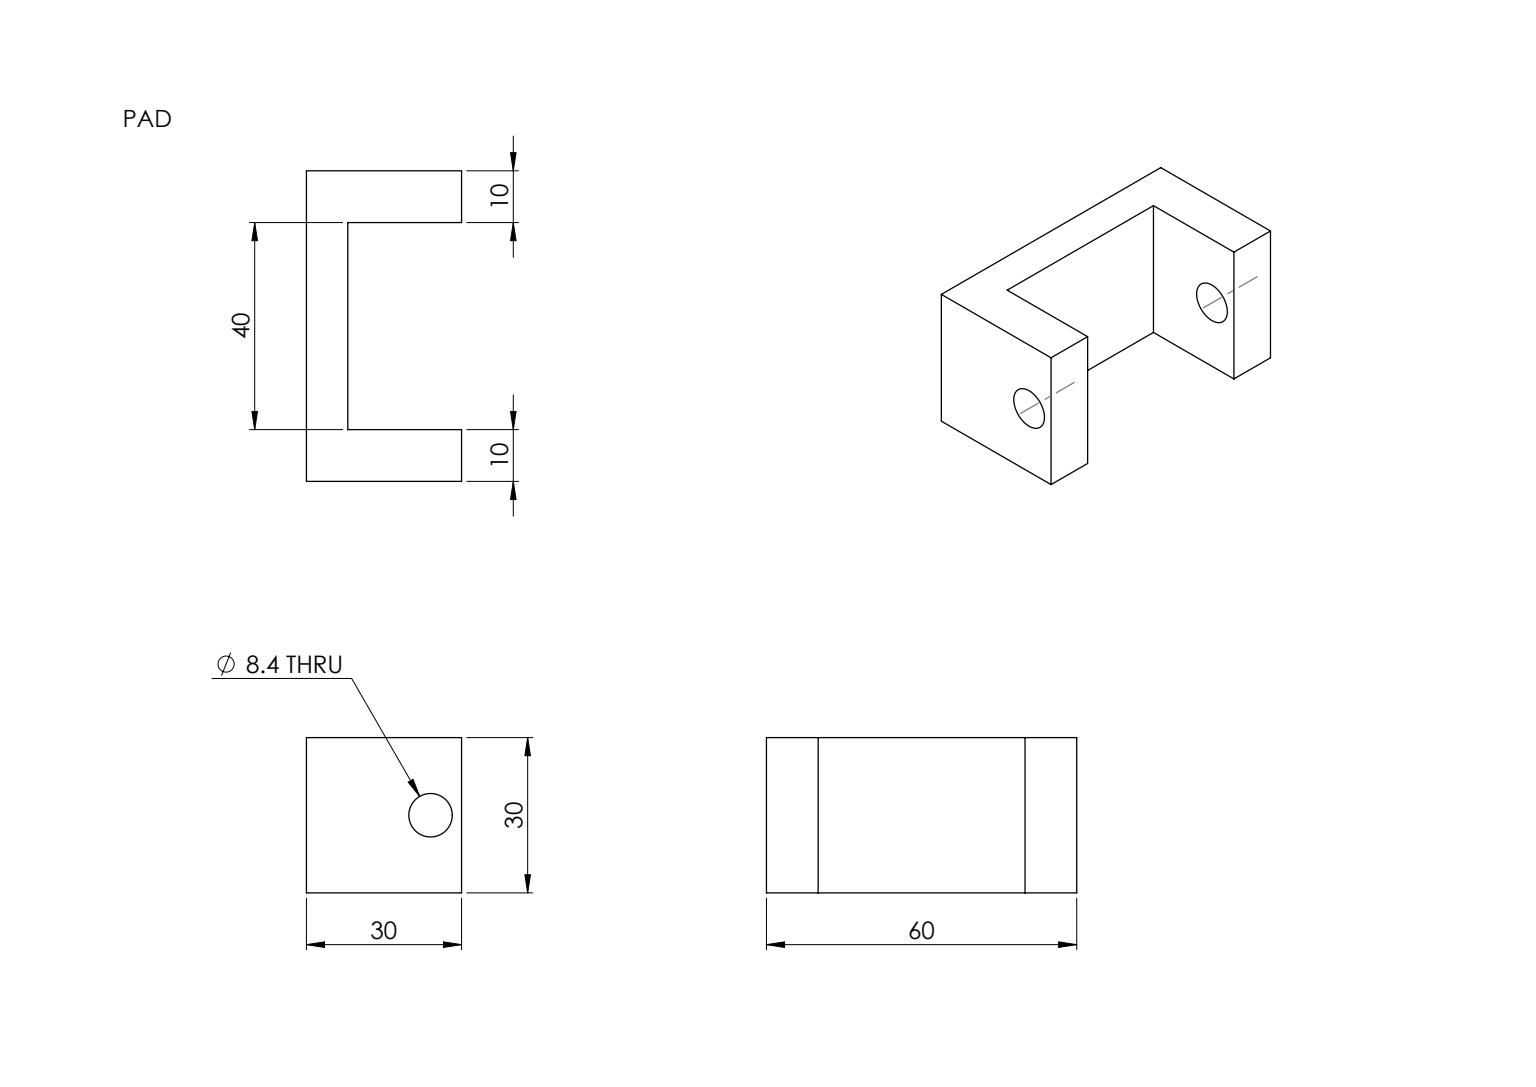
ISO-10303-21;
HEADER;
FILE_DESCRIPTION (('STEP AP214'),
    '1' );
FILE_NAME ('pad.step',
    '2026-10-08T07:58:12',
    ( '' ),
    ( '' ),
    'SwSTEP 2.0',
    'SolidWorks 2026',
    '' );
FILE_SCHEMA (( 'AUTOMOTIVE_DESIGN' ));
ENDSEC;

DATA;
#173=AXIS2_PLACEMENT_3D ( 'NONE', #29896, #20170, #1948 ) ;
#224=DIRECTION ( 'NONE',  ( -2.312964634635740985E-16, 1.000000000000000000, 0.000000000000000000 ) ) ;
#231=DIRECTION ( 'NONE',  ( -1.000000000000000000, 0.000000000000000000, -0.000000000000000000 ) ) ;
#282=APPLICATION_CONTEXT ( 'automotive_design' ) ;
#429=DIRECTION ( 'NONE',  ( -1.000000000000000000, 0.000000000000000000, 0.000000000000000000 ) ) ;
#437=CARTESIAN_POINT ( 'NONE',  ( 58.50000000000001421, -88.00000000000000000, -30.00000000000000000 ) ) ;
#514=PRODUCT_CONTEXT ( 'NONE', #30526, 'mechanical' ) ;
#517=DIRECTION ( 'NONE',  ( -0.000000000000000000, -0.000000000000000000, -1.000000000000000000 ) ) ;
#527=DIRECTION ( 'NONE',  ( 0.000000000000000000, -1.000000000000000000, 0.000000000000000000 ) ) ;
#576=VERTEX_POINT ( 'NONE', #31507 ) ;
#618=AXIS2_PLACEMENT_3D ( 'NONE', #25395, #27609, #7178 ) ;
#690=FACE_BOUND ( 'NONE', #27435, .T. ) ;
#731=AXIS2_PLACEMENT_3D ( 'NONE', #2930, #31053, #13311 ) ;
#790=UNCERTAINTY_MEASURE_WITH_UNIT (LENGTH_MEASURE( 1.000000000000000082E-05 ), #19917, 'distance_accuracy_value', 'NONE');
#873=DIRECTION ( 'NONE',  ( 0.000000000000000000, -1.000000000000000000, 0.000000000000000000 ) ) ;
#909=VECTOR ( 'NONE', #224, 1000.000000000000000 ) ;
#925=DIRECTION ( 'NONE',  ( 0.000000000000000000, 0.000000000000000000, -1.000000000000000000 ) ) ;
#942=LINE ( 'NONE', #11680, #28706 ) ;
#1001=( NAMED_UNIT ( * ) PLANE_ANGLE_UNIT ( ) SI_UNIT ( $, .RADIAN. ) );
#1029=LINE ( 'NONE', #22776, #23544 ) ;
#1286=ORIENTED_EDGE ( 'NONE', *, *, #8935, .F. ) ;
#1306=DIRECTION ( 'NONE',  ( 0.000000000000000000, 0.000000000000000000, -1.000000000000000000 ) ) ;
#1476=ADVANCED_FACE ( 'NONE', ( #27189 ), #19854, .F. ) ;
#1731=ORIENTED_EDGE ( 'NONE', *, *, #24172, .F. ) ;
#1733=CARTESIAN_POINT ( 'NONE',  ( 64.50000000000000000, 0.000000000000000000, 30.00000000000000000 ) ) ;
#1853=EDGE_CURVE ( 'NONE', #10439, #8233, #21818, .T. ) ;
#1857=MECHANICAL_DESIGN_GEOMETRIC_PRESENTATION_REPRESENTATION('',(#32884),#26900);
#1873=ORIENTED_EDGE ( 'NONE', *, *, #10837, .T. ) ;
#1914=LINE ( 'NONE', #1733, #4519 ) ;
#1938=DIRECTION ( 'NONE',  ( -2.312964634635740985E-16, 1.000000000000000000, 0.000000000000000000 ) ) ;
#1948=DIRECTION ( 'NONE',  ( -1.000000000000000000, 0.000000000000000000, 0.000000000000000000 ) ) ;
#2049=EDGE_LOOP ( 'NONE', ( #24718, #18953, #9756, #29271 ) ) ;
#2299=VERTEX_POINT ( 'NONE', #7168 ) ;
#2404=AXIS2_PLACEMENT_3D ( 'NONE', #8872, #11941, #4266 ) ;
#2667=LINE ( 'NONE', #7776, #31465 ) ;
#2693=CIRCLE ( 'NONE', #19527, 4.200000000000001954 ) ;
#2728=VERTEX_POINT ( 'NONE', #14113 ) ;
#2741=ADVANCED_BREP_SHAPE_REPRESENTATION ( '', ( #23155, #2404 ), #13844 ) ;
#2787=FACE_OUTER_BOUND ( 'NONE', #5141, .T. ) ;
#2913=VECTOR ( 'NONE', #28866, 1000.000000000000000 ) ;
#2915=CARTESIAN_POINT ( 'NONE',  ( 64.50000000000000000, 0.000000000000000000, -30.00000000000000000 ) ) ;
#2930=CARTESIAN_POINT ( 'NONE',  ( 64.50000000000000000, 0.000000000000000000, -30.00000000000000000 ) ) ;
#2935=ORIENTED_EDGE ( 'NONE', *, *, #16237, .F. ) ;
#2937=DIRECTION ( 'NONE',  ( -0.000000000000000000, -0.000000000000000000, -1.000000000000000000 ) ) ;
#2976=DIRECTION ( 'NONE',  ( -1.000000000000000000, 0.000000000000000000, 0.000000000000000000 ) ) ;
#3040=ORIENTED_EDGE ( 'NONE', *, *, #16988, .T. ) ;
#3111=ORIENTED_EDGE ( 'NONE', *, *, #30533, .F. ) ;
#3168=VERTEX_POINT ( 'NONE', #4394 ) ;
#3249=ORIENTED_EDGE ( 'NONE', *, *, #12805, .F. ) ;
#3324=ADVANCED_FACE ( 'NONE', ( #15125 ), #7471, .T. ) ;
#3411=DIRECTION ( 'NONE',  ( 0.000000000000000000, -1.000000000000000000, 0.000000000000000000 ) ) ;
#3539=CARTESIAN_POINT ( 'NONE',  ( 64.50000000000000000, -73.00000000000000000, -20.00000000000000000 ) ) ;
#3569=DIRECTION ( 'NONE',  ( -1.000000000000000000, 0.000000000000000000, -0.000000000000000000 ) ) ;
#3583=CYLINDRICAL_SURFACE ( 'NONE', #25243, 4.200000000000001954 ) ;
#3875=EDGE_CURVE ( 'NONE', #2728, #26702, #9594, .T. ) ;
#4080=( NAMED_UNIT ( * ) PLANE_ANGLE_UNIT ( ) SI_UNIT ( $, .RADIAN. ) );
#4152=ADVANCED_FACE ( 'NONE', ( #2787, #15720 ), #16050, .F. ) ;
#4238=FACE_BOUND ( 'NONE', #23300, .T. ) ;
#4250=AXIS2_PLACEMENT_3D ( 'NONE', #26142, #26305, #2976 ) ;
#4266=DIRECTION ( 'NONE',  ( 1.000000000000000000, 0.000000000000000000, 0.000000000000000000 ) ) ;
#4343=LINE ( 'NONE', #12347, #9410 ) ;
#4347=ORIENTED_EDGE ( 'NONE', *, *, #33290, .F. ) ;
#4378=EDGE_LOOP ( 'NONE', ( #20165, #13924, #27388, #19802 ) ) ;
#4394=CARTESIAN_POINT ( 'NONE',  ( 62.70000000000001705, -88.00000000000000000, 20.00000000000000000 ) ) ;
#4434=AXIS2_PLACEMENT_3D ( 'NONE', #13167, #31559, #231 ) ;
#4473=VERTEX_POINT ( 'NONE', #16883 ) ;
#4519=VECTOR ( 'NONE', #22349, 1000.000000000000000 ) ;
#4562=ADVANCED_FACE ( 'NONE', ( #22847 ), #32721, .F. ) ;
#4581=CARTESIAN_POINT ( 'NONE',  ( 64.50000000000000000, -73.00000000000000000, 20.00000000000000000 ) ) ;
#4635=DIRECTION ( 'NONE',  ( -0.000000000000000000, -0.000000000000000000, -1.000000000000000000 ) ) ;
#4744=ADVANCED_FACE ( 'NONE', ( #33061 ), #17222, .T. ) ;
#4781=AXIS2_PLACEMENT_3D ( 'NONE', #9687, #19741, #6970 ) ;
#4857=CARTESIAN_POINT ( 'NONE',  ( 4.764707147349631625E-14, -103.0000000000000284, 20.00000000000000000 ) ) ;
#5031=DIRECTION ( 'NONE',  ( -0.000000000000000000, -0.000000000000000000, -1.000000000000000000 ) ) ;
#5041=LINE ( 'NONE', #7432, #22790 ) ;
#5141=EDGE_LOOP ( 'NONE', ( #18509, #5550, #27056, #19591 ) ) ;
#5167=LINE ( 'NONE', #17775, #11213 ) ;
#5313=ORIENTED_EDGE ( 'NONE', *, *, #3875, .T. ) ;
#5478=FACE_OUTER_BOUND ( 'NONE', #15118, .T. ) ;
#5512=EDGE_LOOP ( 'NONE', ( #20983, #9749, #20862, #21763 ) ) ;
#5550=ORIENTED_EDGE ( 'NONE', *, *, #1853, .F. ) ;
#5623=EDGE_CURVE ( 'NONE', #4473, #30739, #9974, .T. ) ;
#5762=VERTEX_POINT ( 'NONE', #17800 ) ;
#5763=LINE ( 'NONE', #8339, #17293 ) ;
#5804=ORIENTED_EDGE ( 'NONE', *, *, #7261, .T. ) ;
#5983=EDGE_CURVE ( 'NONE', #8169, #8276, #19476, .T. ) ;
#6103=SHAPE_DEFINITION_REPRESENTATION ( #24933, #12832 ) ;
#6268=ORIENTED_EDGE ( 'NONE', *, *, #33328, .F. ) ;
#6393=LINE ( 'NONE', #11510, #11291 ) ;
#6521=CIRCLE ( 'NONE', #14123, 4.200000000000001954 ) ;
#6734=DIRECTION ( 'NONE',  ( 2.312964634635740985E-16, -1.000000000000000000, 0.000000000000000000 ) ) ;
#6750=VECTOR ( 'NONE', #517, 1000.000000000000000 ) ;
#6970=DIRECTION ( 'NONE',  ( 1.000000000000000000, 0.000000000000000000, 0.000000000000000000 ) ) ;
#6994=EDGE_CURVE ( 'NONE', #13849, #25466, #5041, .T. ) ;
#7168=CARTESIAN_POINT ( 'NONE',  ( 34.49999999999999289, -72.99999999999998579, 30.00000000000000000 ) ) ;
#7178=DIRECTION ( 'NONE',  ( 1.000000000000000000, 0.000000000000000000, 0.000000000000000000 ) ) ;
#7248=ORIENTED_EDGE ( 'NONE', *, *, #14578, .T. ) ;
#7261=EDGE_CURVE ( 'NONE', #13192, #9072, #2693, .T. ) ;
#7432=CARTESIAN_POINT ( 'NONE',  ( 124.9999999999999716, -73.00000000000002842, -20.00000000000000000 ) ) ;
#7471=PLANE ( 'NONE',  #25623 ) ;
#7600=CARTESIAN_POINT ( 'NONE',  ( 34.49999999999999289, -72.99999999999998579, 30.00000000000000000 ) ) ;
#7609=CARTESIAN_POINT ( 'NONE',  ( 42.49999999999999289, -72.99999999999998579, -20.00000000000000000 ) ) ;
#7633=DIRECTION ( 'NONE',  ( -0.000000000000000000, -0.000000000000000000, 1.000000000000000000 ) ) ;
#7739=AXIS2_PLACEMENT_3D ( 'NONE', #17395, #30007, #20287 ) ;
#7761=LINE ( 'NONE', #23428, #2913 ) ;
#7776=CARTESIAN_POINT ( 'NONE',  ( 64.50000000000000000, -73.00000000000000000, 30.00000000000000000 ) ) ;
#7879=VERTEX_POINT ( 'NONE', #26448 ) ;
#7921=DIRECTION ( 'NONE',  ( 1.000000000000000000, -4.625929269271484928E-16, 0.000000000000000000 ) ) ;
#8163=AXIS2_PLACEMENT_3D ( 'NONE', #19746, #27412, #3569 ) ;
#8169=VERTEX_POINT ( 'NONE', #9396 ) ;
#8233=VERTEX_POINT ( 'NONE', #19792 ) ;
#8276=VERTEX_POINT ( 'NONE', #28478 ) ;
#8339=CARTESIAN_POINT ( 'NONE',  ( 42.50000000000000000, -103.0000000000000142, -51.04834939252008041 ) ) ;
#8376=DIRECTION ( 'NONE',  ( -1.000000000000000000, 0.000000000000000000, 0.000000000000000000 ) ) ;
#8538=CARTESIAN_POINT ( 'NONE',  ( -3.376928366568182163E-14, -72.99999999999997158, 20.00000000000000000 ) ) ;
#8675=LINE ( 'NONE', #19067, #6750 ) ;
#8699=FACE_OUTER_BOUND ( 'NONE', #20171, .T. ) ;
#8824=( NAMED_UNIT ( * ) SI_UNIT ( $, .STERADIAN. ) SOLID_ANGLE_UNIT ( ) );
#8872=CARTESIAN_POINT ( 'NONE',  ( 0.000000000000000000, 0.000000000000000000, 0.000000000000000000 ) ) ;
#8879=ADVANCED_FACE ( 'NONE', ( #4238, #19581 ), #17018, .F. ) ;
#8935=EDGE_CURVE ( 'NONE', #8276, #8169, #6521, .T. ) ;
#9061=LINE ( 'NONE', #32909, #18707 ) ;
#9072=VERTEX_POINT ( 'NONE', #15767 ) ;
#9151=VERTEX_POINT ( 'NONE', #16768 ) ;
#9362=ORIENTED_EDGE ( 'NONE', *, *, #12805, .T. ) ;
#9396=CARTESIAN_POINT ( 'NONE',  ( 62.70000000000001705, -88.00000000000000000, -30.00000000000000000 ) ) ;
#9402=EDGE_CURVE ( 'NONE', #27639, #28972, #27107, .T. ) ;
#9410=VECTOR ( 'NONE', #20356, 1000.000000000000000 ) ;
#9434=VECTOR ( 'NONE', #3411, 1000.000000000000000 ) ;
#9594=LINE ( 'NONE', #28169, #16391 ) ;
#9672=( NAMED_UNIT ( * ) SI_UNIT ( $, .STERADIAN. ) SOLID_ANGLE_UNIT ( ) );
#9687=CARTESIAN_POINT ( 'NONE',  ( 58.50000000000001421, -88.00000000000000000, 30.00000000000000000 ) ) ;
#9707=PRODUCT ( 'pad', 'pad', '', ( #514 ) ) ;
#9749=ORIENTED_EDGE ( 'NONE', *, *, #15399, .F. ) ;
#9756=ORIENTED_EDGE ( 'NONE', *, *, #30533, .T. ) ;
#9836=CARTESIAN_POINT ( 'NONE',  ( 4.764707147349631625E-14, -103.0000000000000284, 30.00000000000000000 ) ) ;
#9850=CARTESIAN_POINT ( 'NONE',  ( 34.49999999999997868, 7.979727989493303168E-15, 30.00000000000000000 ) ) ;
#9851=PRESENTATION_STYLE_ASSIGNMENT (( #25517 ) ) ;
#9916=LINE ( 'NONE', #23373, #11098 ) ;
#9974=LINE ( 'NONE', #4857, #31993 ) ;
#10163=DIRECTION ( 'NONE',  ( -0.000000000000000000, -0.000000000000000000, -1.000000000000000000 ) ) ;
#10168=EDGE_CURVE ( 'NONE', #21673, #30739, #5763, .T. ) ;
#10180=VERTEX_POINT ( 'NONE', #21603 ) ;
#10439=VERTEX_POINT ( 'NONE', #14616 ) ;
#10563=ORIENTED_EDGE ( 'NONE', *, *, #15365, .F. ) ;
#10644=ADVANCED_FACE ( 'NONE', ( #28749 ), #31137, .T. ) ;
#10664=DIRECTION ( 'NONE',  ( 1.000000000000000000, -4.625929269271484928E-16, 0.000000000000000000 ) ) ;
#10691=DIRECTION ( 'NONE',  ( -1.000000000000000000, 0.000000000000000000, 0.000000000000000000 ) ) ;
#10759=CARTESIAN_POINT ( 'NONE',  ( 0.000000000000000000, 0.000000000000000000, -30.00000000000000000 ) ) ;
#10761=ADVANCED_FACE ( 'NONE', ( #15956 ), #26184, .T. ) ;
#10837=EDGE_CURVE ( 'NONE', #3168, #9151, #13223, .T. ) ;
#10927=DIRECTION ( 'NONE',  ( -1.000000000000000000, 0.000000000000000000, -0.000000000000000000 ) ) ;
#10940=LINE ( 'NONE', #23876, #16445 ) ;
#11052=ORIENTED_EDGE ( 'NONE', *, *, #18559, .F. ) ;
#11057=VECTOR ( 'NONE', #13458, 1000.000000000000000 ) ;
#11098=VECTOR ( 'NONE', #4635, 1000.000000000000000 ) ;
#11213=VECTOR ( 'NONE', #1938, 1000.000000000000000 ) ;
#11291=VECTOR ( 'NONE', #29908, 1000.000000000000000 ) ;
#11348=ORIENTED_EDGE ( 'NONE', *, *, #28931, .T. ) ;
#11427=EDGE_LOOP ( 'NONE', ( #17978, #32147, #14905, #2935, #25416, #24673, #1731, #4347 ) ) ;
#11461=ORIENTED_EDGE ( 'NONE', *, *, #33328, .T. ) ;
#11510=CARTESIAN_POINT ( 'NONE',  ( 124.9999999999999716, -73.00000000000002842, -30.00000000000000000 ) ) ;
#11680=CARTESIAN_POINT ( 'NONE',  ( 42.49999999999998579, 9.830099697201894772E-15, 20.00000000000000000 ) ) ;
#11941=DIRECTION ( 'NONE',  ( 0.000000000000000000, 0.000000000000000000, 1.000000000000000000 ) ) ;
#12002=CARTESIAN_POINT ( 'NONE',  ( 58.50000000000001421, -88.00000000000000000, -30.00000000000000000 ) ) ;
#12160=CARTESIAN_POINT ( 'NONE',  ( 42.49999999999999289, -103.0000000000000142, -20.00000000000000000 ) ) ;
#12307=CIRCLE ( 'NONE', #21020, 4.200000000000001954 ) ;
#12314=CLOSED_SHELL ( 'NONE', ( #19715, #4562, #4152, #10644, #23936, #10761, #3324, #15148, #4744, #19588, #22933, #8879, #1476, #17501 ) ) ;
#12336=STYLED_ITEM ( 'NONE', ( #14469 ), #23155 ) ;
#12347=CARTESIAN_POINT ( 'NONE',  ( 62.70000000000001705, -88.00000000000000000, -30.00000000000000000 ) ) ;
#12474=ORIENTED_EDGE ( 'NONE', *, *, #12848, .T. ) ;
#12573=DIRECTION ( 'NONE',  ( -1.000000000000000000, 4.625929269271484928E-16, 0.000000000000000000 ) ) ;
#12662=DIRECTION ( 'NONE',  ( 0.000000000000000000, 0.000000000000000000, -1.000000000000000000 ) ) ;
#12742=DIRECTION ( 'NONE',  ( -1.000000000000000000, -2.312964634635740985E-16, 0.000000000000000000 ) ) ;
#12744=( LENGTH_UNIT ( ) NAMED_UNIT ( * ) SI_UNIT ( .MILLI., .METRE. ) );
#12805=EDGE_CURVE ( 'NONE', #9151, #7879, #16672, .T. ) ;
#12832=SHAPE_REPRESENTATION ( 'pad', ( #2404 ), #13844 ) ;
#12848=EDGE_CURVE ( 'NONE', #13192, #8276, #8675, .T. ) ;
#12936=ORIENTED_EDGE ( 'NONE', *, *, #10837, .F. ) ;
#13063=ORIENTED_EDGE ( 'NONE', *, *, #5983, .T. ) ;
#13162=CARTESIAN_POINT ( 'NONE',  ( 34.49999999999998579, -2.093232994345345860E-14, -30.00000000000000000 ) ) ;
#13167=CARTESIAN_POINT ( 'NONE',  ( 0.000000000000000000, 0.000000000000000000, 30.00000000000000000 ) ) ;
#13192=VERTEX_POINT ( 'NONE', #31318 ) ;
#13223=CIRCLE ( 'NONE', #25753, 4.200000000000001954 ) ;
#13307=UNCERTAINTY_MEASURE_WITH_UNIT (LENGTH_MEASURE( 1.000000000000000082E-05 ), #32499, 'distance_accuracy_value', 'NONE');
#13311=DIRECTION ( 'NONE',  ( 0.000000000000000000, 0.000000000000000000, 1.000000000000000000 ) ) ;
#13458=DIRECTION ( 'NONE',  ( 0.000000000000000000, 0.000000000000000000, 1.000000000000000000 ) ) ;
#13482=ORIENTED_EDGE ( 'NONE', *, *, #5623, .T. ) ;
#13525=VECTOR ( 'NONE', #16707, 1000.000000000000000 ) ;
#13630=DIRECTION ( 'NONE',  ( 0.000000000000000000, 0.000000000000000000, -1.000000000000000000 ) ) ;
#13676=VERTEX_POINT ( 'NONE', #19358 ) ;
#13680=EDGE_LOOP ( 'NONE', ( #32271, #17127, #30068, #7248 ) ) ;
#13750=CIRCLE ( 'NONE', #173, 4.200000000000001954 ) ;
#13785=DIRECTION ( 'NONE',  ( -0.000000000000000000, -0.000000000000000000, 1.000000000000000000 ) ) ;
#13844=( GEOMETRIC_REPRESENTATION_CONTEXT ( 3 ) GLOBAL_UNCERTAINTY_ASSIGNED_CONTEXT ( ( #13307 ) ) GLOBAL_UNIT_ASSIGNED_CONTEXT ( ( #32499, #1001, #8824 ) ) REPRESENTATION_CONTEXT ( 'NONE', 'WORKASPACE' ) );
#13849=VERTEX_POINT ( 'NONE', #7609 ) ;
#13888=ORIENTED_EDGE ( 'NONE', *, *, #3875, .F. ) ;
#13924=ORIENTED_EDGE ( 'NONE', *, *, #31036, .F. ) ;
#14110=FILL_AREA_STYLE_COLOUR ( '', #16538 ) ;
#14113=CARTESIAN_POINT ( 'NONE',  ( 64.50000000000000000, -103.0000000000000000, -30.00000000000000000 ) ) ;
#14123=AXIS2_PLACEMENT_3D ( 'NONE', #437, #21048, #14973 ) ;
#14303=SURFACE_SIDE_STYLE ('',( #17371 ) ) ;
#14375=CARTESIAN_POINT ( 'NONE',  ( 42.50000000000000000, -103.0000000000000142, 20.00000000000000355 ) ) ;
#14396=DIRECTION ( 'NONE',  ( -0.000000000000000000, -0.000000000000000000, -1.000000000000000000 ) ) ;
#14469=PRESENTATION_STYLE_ASSIGNMENT (( #24704 ) ) ;
#14533=EDGE_CURVE ( 'NONE', #28972, #4473, #10940, .T. ) ;
#14578=EDGE_CURVE ( 'NONE', #10439, #4473, #21316, .T. ) ;
#14616=CARTESIAN_POINT ( 'NONE',  ( 64.50000000000000000, -103.0000000000000000, 30.00000000000000000 ) ) ;
#14759=DIRECTION ( 'NONE',  ( 4.625929269271485914E-16, -1.000000000000000000, 0.000000000000000000 ) ) ;
#14802=ORIENTED_EDGE ( 'NONE', *, *, #7261, .F. ) ;
#14806=( NAMED_UNIT ( * ) SI_UNIT ( $, .STERADIAN. ) SOLID_ANGLE_UNIT ( ) );
#14905=ORIENTED_EDGE ( 'NONE', *, *, #9402, .F. ) ;
#14973=DIRECTION ( 'NONE',  ( -1.000000000000000000, 0.000000000000000000, 0.000000000000000000 ) ) ;
#15099=AXIS2_PLACEMENT_3D ( 'NONE', #18525, #31791, #19183 ) ;
#15104=DIRECTION ( 'NONE',  ( 1.000000000000000000, 4.625929269271485914E-16, 0.000000000000000000 ) ) ;
#15118=EDGE_LOOP ( 'NONE', ( #26429, #13888, #3111, #28199 ) ) ;
#15125=FACE_OUTER_BOUND ( 'NONE', #11427, .T. ) ;
#15148=ADVANCED_FACE ( 'NONE', ( #19857, #33154 ), #27523, .T. ) ;
#15365=EDGE_CURVE ( 'NONE', #9072, #13192, #13750, .T. ) ;
#15399=EDGE_CURVE ( 'NONE', #26702, #21673, #22561, .T. ) ;
#15467=SURFACE_SIDE_STYLE ('',( #17681 ) ) ;
#15629=CARTESIAN_POINT ( 'NONE',  ( -3.376928366568182163E-14, -72.99999999999997158, 30.00000000000000000 ) ) ;
#15640=EDGE_CURVE ( 'NONE', #2728, #5762, #18292, .T. ) ;
#15720=FACE_BOUND ( 'NONE', #17974, .T. ) ;
#15732=DIRECTION ( 'NONE',  ( -1.000000000000000000, -4.625929269271485914E-16, 0.000000000000000000 ) ) ;
#15767=CARTESIAN_POINT ( 'NONE',  ( 62.70000000000001705, -88.00000000000000000, -20.00000000000000000 ) ) ;
#15866=PLANE ( 'NONE',  #731 ) ;
#15956=FACE_OUTER_BOUND ( 'NONE', #13680, .T. ) ;
#16050=PLANE ( 'NONE',  #4434 ) ;
#16071=LINE ( 'NONE', #20693, #22490 ) ;
#16115=AXIS2_PLACEMENT_3D ( 'NONE', #10759, #13630, #10927 ) ;
#16156=DIRECTION ( 'NONE',  ( 0.000000000000000000, 0.000000000000000000, 1.000000000000000000 ) ) ;
#16237=EDGE_CURVE ( 'NONE', #13849, #27639, #9061, .T. ) ;
#16391=VECTOR ( 'NONE', #20157, 1000.000000000000000 ) ;
#16433=EDGE_CURVE ( 'NONE', #8233, #5762, #9916, .T. ) ;
#16445=VECTOR ( 'NONE', #873, 1000.000000000000000 ) ;
#16538=COLOUR_RGB ( '', 0.09019608, 0.27058824, 0.51372549) ;
#16672=LINE ( 'NONE', #27069, #20914 ) ;
#16707=DIRECTION ( 'NONE',  ( -1.000000000000000000, -4.625929269271485914E-16, 0.000000000000000000 ) ) ;
#16768=CARTESIAN_POINT ( 'NONE',  ( 54.30000000000001137, -88.00000000000000000, 20.00000000000000000 ) ) ;
#16883=CARTESIAN_POINT ( 'NONE',  ( 64.50000000000000000, -103.0000000000000000, 20.00000000000000000 ) ) ;
#16988=EDGE_CURVE ( 'NONE', #21673, #13849, #1029, .T. ) ;
#17018=PLANE ( 'NONE',  #8163 ) ;
#17027=FILL_AREA_STYLE ('',( #27420 ) ) ;
#17105=CARTESIAN_POINT ( 'NONE',  ( 58.50000000000001421, -88.00000000000000000, 20.00000000000000000 ) ) ;
#17119=FACE_OUTER_BOUND ( 'NONE', #23530, .T. ) ;
#17127=ORIENTED_EDGE ( 'NONE', *, *, #29739, .F. ) ;
#17166=ORIENTED_EDGE ( 'NONE', *, *, #5983, .F. ) ;
#17222=PLANE ( 'NONE',  #7739 ) ;
#17286=PRODUCT_DEFINITION ( 'UNKNOWN', '', #26254, #18513 ) ;
#17293=VECTOR ( 'NONE', #16156, 1000.000000000000000 ) ;
#17308=DIRECTION ( 'NONE',  ( -1.000000000000000000, 0.000000000000000000, -0.000000000000000000 ) ) ;
#17371=SURFACE_STYLE_FILL_AREA ( #17027 ) ;
#17395=CARTESIAN_POINT ( 'NONE',  ( 42.49999999999999289, -72.99999999999998579, -51.04834939252008041 ) ) ;
#17501=ADVANCED_FACE ( 'NONE', ( #17119 ), #33297, .F. ) ;
#17550=AXIS2_PLACEMENT_3D ( 'NONE', #22412, #1306, #17308 ) ;
#17619=DIRECTION ( 'NONE',  ( -1.000000000000000000, -4.625929269271485914E-16, 0.000000000000000000 ) ) ;
#17680=DIRECTION ( 'NONE',  ( 2.312964634635740985E-16, -1.000000000000000000, 0.000000000000000000 ) ) ;
#17681=SURFACE_STYLE_FILL_AREA ( #24504 ) ;
#17775=CARTESIAN_POINT ( 'NONE',  ( 34.49999999999997868, 7.979727989493303168E-15, 30.00000000000000000 ) ) ;
#17800=CARTESIAN_POINT ( 'NONE',  ( 34.50000000000000000, -103.0000000000000142, -30.00000000000000000 ) ) ;
#17974=EDGE_LOOP ( 'NONE', ( #20146, #24747 ) ) ;
#17978=ORIENTED_EDGE ( 'NONE', *, *, #18891, .T. ) ;
#18084=EDGE_LOOP ( 'NONE', ( #33426, #31262, #28653, #3040 ) ) ;
#18266=EDGE_CURVE ( 'NONE', #576, #10439, #1914, .T. ) ;
#18292=LINE ( 'NONE', #33459, #21359 ) ;
#18386=ORIENTED_EDGE ( 'NONE', *, *, #21820, .F. ) ;
#18501=ORIENTED_EDGE ( 'NONE', *, *, #24317, .F. ) ;
#18509=ORIENTED_EDGE ( 'NONE', *, *, #21939, .F. ) ;
#18513=PRODUCT_DEFINITION_CONTEXT ( 'detailed design', #282, 'design' ) ;
#18525=CARTESIAN_POINT ( 'NONE',  ( 64.50000000000000000, 0.000000000000000000, 30.00000000000000000 ) ) ;
#18559=EDGE_CURVE ( 'NONE', #9072, #8169, #4343, .T. ) ;
#18707=VECTOR ( 'NONE', #33074, 1000.000000000000000 ) ;
#18816=CARTESIAN_POINT ( 'NONE',  ( 58.50000000000001421, -88.00000000000000000, -20.00000000000000000 ) ) ;
#18891=EDGE_CURVE ( 'NONE', #2299, #576, #16071, .T. ) ;
#18953=ORIENTED_EDGE ( 'NONE', *, *, #24172, .T. ) ;
#19067=CARTESIAN_POINT ( 'NONE',  ( 54.30000000000001137, -88.00000000000000000, -30.00000000000000000 ) ) ;
#19074=CARTESIAN_POINT ( 'NONE',  ( 64.50000000000000000, -73.00000000000000000, -30.00000000000000000 ) ) ;
#19183=DIRECTION ( 'NONE',  ( -0.000000000000000000, 0.000000000000000000, -1.000000000000000000 ) ) ;
#19202=VECTOR ( 'NONE', #17619, 1000.000000000000000 ) ;
#19261=EDGE_LOOP ( 'NONE', ( #18501, #19844, #24226, #13482 ) ) ;
#19358=CARTESIAN_POINT ( 'NONE',  ( 34.50000000000000000, -72.99999999999998579, -30.00000000000000000 ) ) ;
#19433=CARTESIAN_POINT ( 'NONE',  ( 4.764707147349631625E-14, -103.0000000000000284, 30.00000000000000000 ) ) ;
#19455=AXIS2_PLACEMENT_3D ( 'NONE', #9850, #12742, #17680 ) ;
#19465=CIRCLE ( 'NONE', #4781, 4.200000000000001954 ) ;
#19476=CIRCLE ( 'NONE', #4250, 4.200000000000001954 ) ;
#19527=AXIS2_PLACEMENT_3D ( 'NONE', #18816, #925, #429 ) ;
#19581=FACE_OUTER_BOUND ( 'NONE', #5512, .T. ) ;
#19588=ADVANCED_FACE ( 'NONE', ( #5478 ), #15866, .F. ) ;
#19591=ORIENTED_EDGE ( 'NONE', *, *, #18891, .F. ) ;
#19594=EDGE_CURVE ( 'NONE', #25466, #26702, #29319, .T. ) ;
#19715=ADVANCED_FACE ( 'NONE', ( #8699 ), #3583, .F. ) ;
#19741=DIRECTION ( 'NONE',  ( -0.000000000000000000, -0.000000000000000000, 1.000000000000000000 ) ) ;
#19746=CARTESIAN_POINT ( 'NONE',  ( 0.000000000000000000, 0.000000000000000000, -20.00000000000000000 ) ) ;
#19792=CARTESIAN_POINT ( 'NONE',  ( 34.50000000000000000, -103.0000000000000142, 30.00000000000000000 ) ) ;
#19802=ORIENTED_EDGE ( 'NONE', *, *, #21939, .T. ) ;
#19839=DIRECTION ( 'NONE',  ( -1.000000000000000000, 0.000000000000000000, 0.000000000000000000 ) ) ;
#19844=ORIENTED_EDGE ( 'NONE', *, *, #9402, .T. ) ;
#19854=CYLINDRICAL_SURFACE ( 'NONE', #33079, 4.200000000000001954 ) ;
#19857=FACE_BOUND ( 'NONE', #25383, .T. ) ;
#19917=( LENGTH_UNIT ( ) NAMED_UNIT ( * ) SI_UNIT ( .MILLI., .METRE. ) );
#20146=ORIENTED_EDGE ( 'NONE', *, *, #28931, .F. ) ;
#20157=DIRECTION ( 'NONE',  ( 0.000000000000000000, 0.000000000000000000, 1.000000000000000000 ) ) ;
#20165=ORIENTED_EDGE ( 'NONE', *, *, #33290, .T. ) ;
#20170=DIRECTION ( 'NONE',  ( 0.000000000000000000, 0.000000000000000000, -1.000000000000000000 ) ) ;
#20171=EDGE_LOOP ( 'NONE', ( #10563, #31079, #13063, #26628 ) ) ;
#20185=DIRECTION ( 'NONE',  ( -1.000000000000000000, -4.625929269271485914E-16, 0.000000000000000000 ) ) ;
#20233=SHAPE_REPRESENTATION_RELATIONSHIP ( 'NONE' , 'NONE' ,  #12832, #2741 ) ;
#20287=DIRECTION ( 'NONE',  ( -2.312964634635740985E-16, 1.000000000000000000, 0.000000000000000000 ) ) ;
#20356=DIRECTION ( 'NONE',  ( -0.000000000000000000, -0.000000000000000000, -1.000000000000000000 ) ) ;
#20512=( GEOMETRIC_REPRESENTATION_CONTEXT ( 3 ) GLOBAL_UNCERTAINTY_ASSIGNED_CONTEXT ( ( #790 ) ) GLOBAL_UNIT_ASSIGNED_CONTEXT ( ( #19917, #4080, #14806 ) ) REPRESENTATION_CONTEXT ( 'NONE', 'WORKASPACE' ) );
#20527=CARTESIAN_POINT ( 'NONE',  ( 64.50000000000000000, -103.0000000000000000, -20.00000000000000000 ) ) ;
#20693=CARTESIAN_POINT ( 'NONE',  ( -3.376928366568182163E-14, -72.99999999999997158, 30.00000000000000000 ) ) ;
#20862=ORIENTED_EDGE ( 'NONE', *, *, #19594, .F. ) ;
#20914=VECTOR ( 'NONE', #13785, 1000.000000000000000 ) ;
#20983=ORIENTED_EDGE ( 'NONE', *, *, #16988, .F. ) ;
#21020=AXIS2_PLACEMENT_3D ( 'NONE', #17105, #12662, #30734 ) ;
#21048=DIRECTION ( 'NONE',  ( -0.000000000000000000, -0.000000000000000000, -1.000000000000000000 ) ) ;
#21139=UNCERTAINTY_MEASURE_WITH_UNIT (LENGTH_MEASURE( 1.000000000000000082E-05 ), #12744, 'distance_accuracy_value', 'NONE');
#21143=VECTOR ( 'NONE', #527, 1000.000000000000000 ) ;
#21316=LINE ( 'NONE', #26933, #29515 ) ;
#21359=VECTOR ( 'NONE', #15732, 1000.000000000000000 ) ;
#21474=FACE_OUTER_BOUND ( 'NONE', #2049, .T. ) ;
#21603=CARTESIAN_POINT ( 'NONE',  ( 64.50000000000000000, -73.00000000000000000, -30.00000000000000000 ) ) ;
#21673=VERTEX_POINT ( 'NONE', #12160 ) ;
#21763=ORIENTED_EDGE ( 'NONE', *, *, #6994, .F. ) ;
#21818=LINE ( 'NONE', #19433, #13525 ) ;
#21820=EDGE_CURVE ( 'NONE', #9151, #3168, #12307, .T. ) ;
#21939=EDGE_CURVE ( 'NONE', #8233, #2299, #5167, .T. ) ;
#22236=ORIENTED_EDGE ( 'NONE', *, *, #15640, .F. ) ;
#22349=DIRECTION ( 'NONE',  ( 0.000000000000000000, -1.000000000000000000, 0.000000000000000000 ) ) ;
#22412=CARTESIAN_POINT ( 'NONE',  ( 0.000000000000000000, 0.000000000000000000, 20.00000000000000000 ) ) ;
#22490=VECTOR ( 'NONE', #7921, 1000.000000000000000 ) ;
#22561=LINE ( 'NONE', #32946, #19202 ) ;
#22600=FACE_OUTER_BOUND ( 'NONE', #30671, .T. ) ;
#22776=CARTESIAN_POINT ( 'NONE',  ( 42.49999999999999289, -72.99999999999998579, -20.00000000000000000 ) ) ;
#22779=PLANE ( 'NONE',  #23809 ) ;
#22790=VECTOR ( 'NONE', #10664, 1000.000000000000000 ) ;
#22847=FACE_OUTER_BOUND ( 'NONE', #28313, .T. ) ;
#22933=ADVANCED_FACE ( 'NONE', ( #690, #21474 ), #26418, .T. ) ;
#23134=( NAMED_UNIT ( * ) PLANE_ANGLE_UNIT ( ) SI_UNIT ( $, .RADIAN. ) );
#23139=DIRECTION ( 'NONE',  ( 4.625929269271484928E-16, 1.000000000000000000, -0.000000000000000000 ) ) ;
#23155=MANIFOLD_SOLID_BREP ( '\X2\00d8\X0\8.4 (8.4) Diameter Hole2', #12314 ) ;
#23156=ORIENTED_EDGE ( 'NONE', *, *, #15365, .T. ) ;
#23255=LINE ( 'NONE', #7600, #27925 ) ;
#23300=EDGE_LOOP ( 'NONE', ( #5804, #23156 ) ) ;
#23373=CARTESIAN_POINT ( 'NONE',  ( 34.50000000000000000, -103.0000000000000142, 30.00000000000000000 ) ) ;
#23428=CARTESIAN_POINT ( 'NONE',  ( 62.70000000000001705, -88.00000000000000000, 30.00000000000000000 ) ) ;
#23459=CARTESIAN_POINT ( 'NONE',  ( 58.50000000000001421, -88.00000000000000000, 30.00000000000000000 ) ) ;
#23530=EDGE_LOOP ( 'NONE', ( #11052, #14802, #12474, #31670 ) ) ;
#23544=VECTOR ( 'NONE', #30783, 1000.000000000000000 ) ;
#23784=VECTOR ( 'NONE', #26759, 1000.000000000000000 ) ;
#23809=AXIS2_PLACEMENT_3D ( 'NONE', #9836, #14759, #15104 ) ;
#23876=CARTESIAN_POINT ( 'NONE',  ( 64.50000000000000000, 0.000000000000000000, 20.00000000000000000 ) ) ;
#23936=ADVANCED_FACE ( 'NONE', ( #22600 ), #22779, .T. ) ;
#24031=CARTESIAN_POINT ( 'NONE',  ( 64.50000000000000000, 0.000000000000000000, -20.00000000000000000 ) ) ;
#24100=ORIENTED_EDGE ( 'NONE', *, *, #1853, .T. ) ;
#24172=EDGE_CURVE ( 'NONE', #13676, #10180, #6393, .T. ) ;
#24226=ORIENTED_EDGE ( 'NONE', *, *, #14533, .T. ) ;
#24317=EDGE_CURVE ( 'NONE', #27639, #30739, #942, .T. ) ;
#24504=FILL_AREA_STYLE ('',( #14110 ) ) ;
#24673=ORIENTED_EDGE ( 'NONE', *, *, #32082, .F. ) ;
#24704=SURFACE_STYLE_USAGE ( .BOTH. , #14303 ) ;
#24718=ORIENTED_EDGE ( 'NONE', *, *, #31036, .T. ) ;
#24747=ORIENTED_EDGE ( 'NONE', *, *, #25967, .F. ) ;
#24933=PRODUCT_DEFINITION_SHAPE ( 'NONE', 'NONE',  #17286 ) ;
#24939=CARTESIAN_POINT ( 'NONE',  ( 42.49999999999999289, -72.99999999999998579, 20.00000000000000000 ) ) ;
#25243=AXIS2_PLACEMENT_3D ( 'NONE', #31702, #29653, #8376 ) ;
#25383=EDGE_LOOP ( 'NONE', ( #12936, #18386 ) ) ;
#25395=CARTESIAN_POINT ( 'NONE',  ( 58.50000000000001421, -88.00000000000000000, 30.00000000000000000 ) ) ;
#25416=ORIENTED_EDGE ( 'NONE', *, *, #6994, .T. ) ;
#25466=VERTEX_POINT ( 'NONE', #3539 ) ;
#25489=CIRCLE ( 'NONE', #30930, 4.200000000000001954 ) ;
#25517=SURFACE_STYLE_USAGE ( .BOTH. , #15467 ) ;
#25623=AXIS2_PLACEMENT_3D ( 'NONE', #15629, #23139, #12573 ) ;
#25753=AXIS2_PLACEMENT_3D ( 'NONE', #32124, #31631, #10691 ) ;
#25938=LINE ( 'NONE', #13162, #909 ) ;
#25967=EDGE_CURVE ( 'NONE', #7879, #29153, #25489, .T. ) ;
#26142=CARTESIAN_POINT ( 'NONE',  ( 58.50000000000001421, -88.00000000000000000, -30.00000000000000000 ) ) ;
#26184=PLANE ( 'NONE',  #15099 ) ;
#26214=ORIENTED_EDGE ( 'NONE', *, *, #10168, .T. ) ;
#26254=PRODUCT_DEFINITION_FORMATION_WITH_SPECIFIED_SOURCE ( 'ANY', '', #9707, .NOT_KNOWN. ) ;
#26305=DIRECTION ( 'NONE',  ( -0.000000000000000000, -0.000000000000000000, -1.000000000000000000 ) ) ;
#26418=PLANE ( 'NONE',  #16115 ) ;
#26429=ORIENTED_EDGE ( 'NONE', *, *, #19594, .T. ) ;
#26448=CARTESIAN_POINT ( 'NONE',  ( 54.30000000000001137, -88.00000000000000000, 30.00000000000000000 ) ) ;
#26535=ORIENTED_EDGE ( 'NONE', *, *, #21820, .T. ) ;
#26581=ORIENTED_EDGE ( 'NONE', *, *, #15399, .T. ) ;
#26628=ORIENTED_EDGE ( 'NONE', *, *, #12848, .F. ) ;
#26702=VERTEX_POINT ( 'NONE', #20527 ) ;
#26759=DIRECTION ( 'NONE',  ( 1.000000000000000000, -4.625929269271484928E-16, 0.000000000000000000 ) ) ;
#26900=( GEOMETRIC_REPRESENTATION_CONTEXT ( 3 ) GLOBAL_UNCERTAINTY_ASSIGNED_CONTEXT ( ( #21139 ) ) GLOBAL_UNIT_ASSIGNED_CONTEXT ( ( #12744, #23134, #9672 ) ) REPRESENTATION_CONTEXT ( 'NONE', 'WORKASPACE' ) );
#26933=CARTESIAN_POINT ( 'NONE',  ( 64.50000000000000000, -103.0000000000000000, 30.00000000000000000 ) ) ;
#27014=COLOUR_RGB ( '', 0.09019608, 0.27058824, 0.51372549) ;
#27056=ORIENTED_EDGE ( 'NONE', *, *, #18266, .F. ) ;
#27069=CARTESIAN_POINT ( 'NONE',  ( 54.30000000000001137, -88.00000000000000000, 30.00000000000000000 ) ) ;
#27107=LINE ( 'NONE', #8538, #23784 ) ;
#27189=FACE_OUTER_BOUND ( 'NONE', #31048, .T. ) ;
#27388=ORIENTED_EDGE ( 'NONE', *, *, #16433, .F. ) ;
#27412=DIRECTION ( 'NONE',  ( 0.000000000000000000, 0.000000000000000000, -1.000000000000000000 ) ) ;
#27420=FILL_AREA_STYLE_COLOUR ( '', #27014 ) ;
#27435=EDGE_LOOP ( 'NONE', ( #1286, #17166 ) ) ;
#27523=PLANE ( 'NONE',  #17550 ) ;
#27609=DIRECTION ( 'NONE',  ( -0.000000000000000000, -0.000000000000000000, 1.000000000000000000 ) ) ;
#27639=VERTEX_POINT ( 'NONE', #24939 ) ;
#27691=DIRECTION ( 'NONE',  ( 1.000000000000000000, 0.000000000000000000, 0.000000000000000000 ) ) ;
#27925=VECTOR ( 'NONE', #5031, 1000.000000000000000 ) ;
#28169=CARTESIAN_POINT ( 'NONE',  ( 64.50000000000000000, -103.0000000000000000, -30.00000000000000000 ) ) ;
#28199=ORIENTED_EDGE ( 'NONE', *, *, #32082, .T. ) ;
#28313=EDGE_LOOP ( 'NONE', ( #1873, #9362, #31946, #6268 ) ) ;
#28478=CARTESIAN_POINT ( 'NONE',  ( 54.30000000000001137, -88.00000000000000000, -30.00000000000000000 ) ) ;
#28653=ORIENTED_EDGE ( 'NONE', *, *, #10168, .F. ) ;
#28706=VECTOR ( 'NONE', #6734, 1000.000000000000000 ) ;
#28749=FACE_OUTER_BOUND ( 'NONE', #4378, .T. ) ;
#28810=LINE ( 'NONE', #2915, #21143 ) ;
#28866=DIRECTION ( 'NONE',  ( -0.000000000000000000, -0.000000000000000000, 1.000000000000000000 ) ) ;
#28931=EDGE_CURVE ( 'NONE', #29153, #7879, #19465, .T. ) ;
#28968=LINE ( 'NONE', #19074, #11057 ) ;
#28972=VERTEX_POINT ( 'NONE', #4581 ) ;
#29153=VERTEX_POINT ( 'NONE', #33536 ) ;
#29271=ORIENTED_EDGE ( 'NONE', *, *, #15640, .T. ) ;
#29319=LINE ( 'NONE', #24031, #9434 ) ;
#29435=ORIENTED_EDGE ( 'NONE', *, *, #14578, .F. ) ;
#29515=VECTOR ( 'NONE', #2937, 1000.000000000000000 ) ;
#29653=DIRECTION ( 'NONE',  ( -0.000000000000000000, -0.000000000000000000, -1.000000000000000000 ) ) ;
#29728=ORIENTED_EDGE ( 'NONE', *, *, #5623, .F. ) ;
#29739=EDGE_CURVE ( 'NONE', #576, #28972, #2667, .T. ) ;
#29741=CARTESIAN_POINT ( 'NONE',  ( 58.50000000000001421, -88.00000000000000000, 30.00000000000000000 ) ) ;
#29896=CARTESIAN_POINT ( 'NONE',  ( 58.50000000000001421, -88.00000000000000000, -20.00000000000000000 ) ) ;
#29908=DIRECTION ( 'NONE',  ( 1.000000000000000000, -4.625929269271484928E-16, 0.000000000000000000 ) ) ;
#30007=DIRECTION ( 'NONE',  ( 1.000000000000000000, 2.312964634635740985E-16, -0.000000000000000000 ) ) ;
#30068=ORIENTED_EDGE ( 'NONE', *, *, #18266, .T. ) ;
#30251=DIRECTION ( 'NONE',  ( -0.000000000000000000, -0.000000000000000000, 1.000000000000000000 ) ) ;
#30526=APPLICATION_CONTEXT ( 'automotive_design' ) ;
#30533=EDGE_CURVE ( 'NONE', #10180, #2728, #28810, .T. ) ;
#30671=EDGE_LOOP ( 'NONE', ( #24100, #32225, #22236, #5313, #26581, #26214, #29728, #29435 ) ) ;
#30734=DIRECTION ( 'NONE',  ( -1.000000000000000000, 0.000000000000000000, 0.000000000000000000 ) ) ;
#30739=VERTEX_POINT ( 'NONE', #14375 ) ;
#30783=DIRECTION ( 'NONE',  ( -2.312964634635740985E-16, 1.000000000000000000, 0.000000000000000000 ) ) ;
#30930=AXIS2_PLACEMENT_3D ( 'NONE', #23459, #7633, #33133 ) ;
#31036=EDGE_CURVE ( 'NONE', #5762, #13676, #25938, .T. ) ;
#31048=EDGE_LOOP ( 'NONE', ( #3249, #26535, #11461, #11348 ) ) ;
#31053=DIRECTION ( 'NONE',  ( -1.000000000000000000, 0.000000000000000000, 0.000000000000000000 ) ) ;
#31079=ORIENTED_EDGE ( 'NONE', *, *, #18559, .T. ) ;
#31137=PLANE ( 'NONE',  #19455 ) ;
#31262=ORIENTED_EDGE ( 'NONE', *, *, #24317, .T. ) ;
#31318=CARTESIAN_POINT ( 'NONE',  ( 54.30000000000001137, -88.00000000000000000, -20.00000000000000000 ) ) ;
#31465=VECTOR ( 'NONE', #10163, 1000.000000000000000 ) ;
#31507=CARTESIAN_POINT ( 'NONE',  ( 64.50000000000000000, -73.00000000000000000, 30.00000000000000000 ) ) ;
#31559=DIRECTION ( 'NONE',  ( 0.000000000000000000, 0.000000000000000000, -1.000000000000000000 ) ) ;
#31631=DIRECTION ( 'NONE',  ( 0.000000000000000000, 0.000000000000000000, -1.000000000000000000 ) ) ;
#31670=ORIENTED_EDGE ( 'NONE', *, *, #8935, .T. ) ;
#31702=CARTESIAN_POINT ( 'NONE',  ( 58.50000000000001421, -88.00000000000000000, -30.00000000000000000 ) ) ;
#31791=DIRECTION ( 'NONE',  ( 1.000000000000000000, 0.000000000000000000, -0.000000000000000000 ) ) ;
#31946=ORIENTED_EDGE ( 'NONE', *, *, #25967, .T. ) ;
#31993=VECTOR ( 'NONE', #20185, 1000.000000000000000 ) ;
#32082=EDGE_CURVE ( 'NONE', #10180, #25466, #28968, .T. ) ;
#32124=CARTESIAN_POINT ( 'NONE',  ( 58.50000000000001421, -88.00000000000000000, 20.00000000000000000 ) ) ;
#32147=ORIENTED_EDGE ( 'NONE', *, *, #29739, .T. ) ;
#32225=ORIENTED_EDGE ( 'NONE', *, *, #16433, .T. ) ;
#32236=AXIS2_PLACEMENT_3D ( 'NONE', #12002, #14396, #19839 ) ;
#32271=ORIENTED_EDGE ( 'NONE', *, *, #14533, .F. ) ;
#32499=( LENGTH_UNIT ( ) NAMED_UNIT ( * ) SI_UNIT ( .MILLI., .METRE. ) );
#32721=CYLINDRICAL_SURFACE ( 'NONE', #618, 4.200000000000001954 ) ;
#32884=STYLED_ITEM ( 'NONE', ( #9851 ), #2741 ) ;
#32909=CARTESIAN_POINT ( 'NONE',  ( 42.49999999999999289, -72.99999999999998579, -51.04834939252008041 ) ) ;
#32946=CARTESIAN_POINT ( 'NONE',  ( 125.0000000000000568, -102.9999999999999716, -20.00000000000000000 ) ) ;
#33021=MECHANICAL_DESIGN_GEOMETRIC_PRESENTATION_REPRESENTATION('',(#12336),#20512);
#33061=FACE_OUTER_BOUND ( 'NONE', #18084, .T. ) ;
#33074=DIRECTION ( 'NONE',  ( 0.000000000000000000, 0.000000000000000000, 1.000000000000000000 ) ) ;
#33079=AXIS2_PLACEMENT_3D ( 'NONE', #29741, #30251, #27691 ) ;
#33133=DIRECTION ( 'NONE',  ( 1.000000000000000000, 0.000000000000000000, 0.000000000000000000 ) ) ;
#33154=FACE_OUTER_BOUND ( 'NONE', #19261, .T. ) ;
#33290=EDGE_CURVE ( 'NONE', #2299, #13676, #23255, .T. ) ;
#33297=CYLINDRICAL_SURFACE ( 'NONE', #32236, 4.200000000000001954 ) ;
#33328=EDGE_CURVE ( 'NONE', #3168, #29153, #7761, .T. ) ;
#33426=ORIENTED_EDGE ( 'NONE', *, *, #16237, .T. ) ;
#33459=CARTESIAN_POINT ( 'NONE',  ( 125.0000000000000568, -102.9999999999999716, -30.00000000000000000 ) ) ;
#33536=CARTESIAN_POINT ( 'NONE',  ( 62.70000000000001705, -88.00000000000000000, 30.00000000000000000 ) ) ;
ENDSEC;
END-ISO-10303-21;
